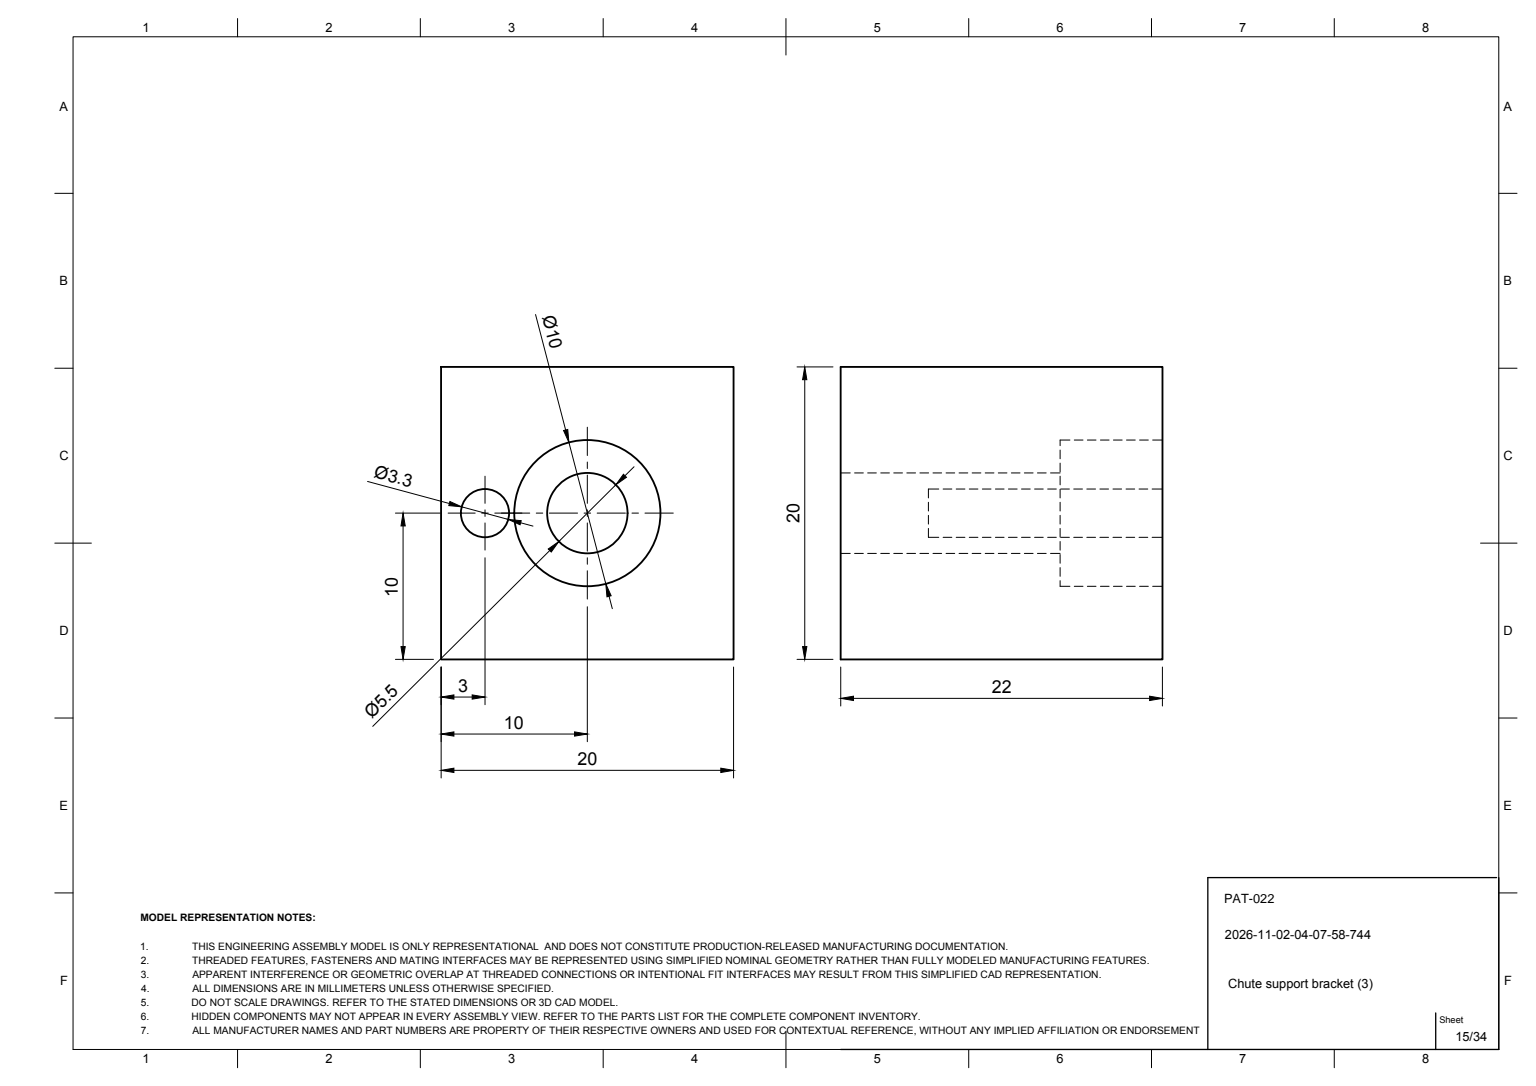
ISO-10303-21;
HEADER;
/* Generated by software containing ST-Developer
 * from STEP Tools, Inc. (www.steptools.com) 
 */

FILE_DESCRIPTION(
/* description */ ('Chute with adjustable gate'),
/* implementation_level */ '2;1');

FILE_NAME(
/* name */ 'Chute support bracket (3).step',
/* time_stamp */ '2026-10-27T10:52:28-07:00',
/* author */ (''),
/* organization */ (''),
/* preprocessor_version */ 'ST-DEVELOPER v20.2',
/* originating_system */ 'Autodesk Translation Framework v15.17.0.0',
/* authorisation */ '');

FILE_SCHEMA (('AUTOMOTIVE_DESIGN { 1 0 10303 214 3 1 1 }'));
ENDSEC;

DATA;
#10=MECHANICAL_DESIGN_GEOMETRIC_PRESENTATION_REPRESENTATION('',(#424),#13094);
#360=SHAPE_REPRESENTATION_RELATIONSHIP('SRR','None',#13261,#392);
#392=ADVANCED_BREP_SHAPE_REPRESENTATION('',(#456),#13070);
#424=STYLED_ITEM('',(#13474),#456);
#456=MANIFOLD_SOLID_BREP('Body1',#7607);
#512=FACE_BOUND('',#1462,.T.);
#513=FACE_BOUND('',#1465,.T.);
#514=FACE_BOUND('',#1468,.T.);
#515=FACE_BOUND('',#1469,.T.);
#660=PLANE('',#8135);
#661=PLANE('',#8139);
#662=PLANE('',#8143);
#663=PLANE('',#8144);
#664=PLANE('',#8145);
#665=PLANE('',#8146);
#666=PLANE('',#8147);
#667=PLANE('',#8148);
#1005=FACE_OUTER_BOUND('',#1458,.T.);
#1006=FACE_OUTER_BOUND('',#1459,.T.);
#1007=FACE_OUTER_BOUND('',#1460,.T.);
#1008=FACE_OUTER_BOUND('',#1461,.T.);
#1009=FACE_OUTER_BOUND('',#1463,.T.);
#1010=FACE_OUTER_BOUND('',#1464,.T.);
#1011=FACE_OUTER_BOUND('',#1466,.T.);
#1012=FACE_OUTER_BOUND('',#1467,.T.);
#1013=FACE_OUTER_BOUND('',#1470,.T.);
#1014=FACE_OUTER_BOUND('',#1471,.T.);
#1015=FACE_OUTER_BOUND('',#1472,.T.);
#1458=EDGE_LOOP('',(#5576,#5577,#5578,#5579));
#1459=EDGE_LOOP('',(#5580));
#1460=EDGE_LOOP('',(#5581,#5582,#5583,#5584));
#1461=EDGE_LOOP('',(#5585));
#1462=EDGE_LOOP('',(#5586));
#1463=EDGE_LOOP('',(#5587,#5588,#5589,#5590));
#1464=EDGE_LOOP('',(#5591,#5592,#5593,#5594));
#1465=EDGE_LOOP('',(#5595));
#1466=EDGE_LOOP('',(#5596,#5597,#5598,#5599));
#1467=EDGE_LOOP('',(#5600,#5601,#5602,#5603));
#1468=EDGE_LOOP('',(#5604));
#1469=EDGE_LOOP('',(#5605));
#1470=EDGE_LOOP('',(#5606,#5607,#5608,#5609));
#1471=EDGE_LOOP('',(#5610,#5611,#5612,#5613));
#1472=EDGE_LOOP('',(#5614,#5615,#5616,#5617));
#2013=LINE('',#11332,#2790);
#2014=LINE('',#11339,#2791);
#2015=LINE('',#11346,#2792);
#2016=LINE('',#11351,#2793);
#2017=LINE('',#11353,#2794);
#2018=LINE('',#11355,#2795);
#2019=LINE('',#11356,#2796);
#2020=LINE('',#11359,#2797);
#2021=LINE('',#11361,#2798);
#2022=LINE('',#11362,#2799);
#2023=LINE('',#11365,#2800);
#2024=LINE('',#11367,#2801);
#2025=LINE('',#11368,#2802);
#2026=LINE('',#11370,#2803);
#2027=LINE('',#11371,#2804);
#2790=VECTOR('',#9147,0.164999999999999);
#2791=VECTOR('',#9156,0.5);
#2792=VECTOR('',#9165,0.274999999999999);
#2793=VECTOR('',#9170,1.);
#2794=VECTOR('',#9171,1.);
#2795=VECTOR('',#9172,1.);
#2796=VECTOR('',#9173,1.);
#2797=VECTOR('',#9176,1.);
#2798=VECTOR('',#9177,1.);
#2799=VECTOR('',#9178,1.);
#2800=VECTOR('',#9181,1.);
#2801=VECTOR('',#9182,1.);
#2802=VECTOR('',#9183,1.);
#2803=VECTOR('',#9186,1.);
#2804=VECTOR('',#9187,1.);
#3456=CIRCLE('',#8133,0.164999999999999);
#3457=CIRCLE('',#8134,0.164999999999999);
#3458=CIRCLE('',#8137,0.5);
#3459=CIRCLE('',#8138,0.5);
#3460=CIRCLE('',#8140,0.274999999999999);
#3461=CIRCLE('',#8142,0.274999999999999);
#3723=VERTEX_POINT('',#11329);
#3724=VERTEX_POINT('',#11331);
#3725=VERTEX_POINT('',#11336);
#3726=VERTEX_POINT('',#11338);
#3727=VERTEX_POINT('',#11342);
#3728=VERTEX_POINT('',#11345);
#3729=VERTEX_POINT('',#11349);
#3730=VERTEX_POINT('',#11350);
#3731=VERTEX_POINT('',#11352);
#3732=VERTEX_POINT('',#11354);
#3733=VERTEX_POINT('',#11358);
#3734=VERTEX_POINT('',#11360);
#3735=VERTEX_POINT('',#11364);
#3736=VERTEX_POINT('',#11366);
#4421=EDGE_CURVE('',#3723,#3723,#3456,.T.);
#4422=EDGE_CURVE('',#3723,#3724,#2013,.T.);
#4423=EDGE_CURVE('',#3724,#3724,#3457,.T.);
#4424=EDGE_CURVE('',#3725,#3725,#3458,.T.);
#4425=EDGE_CURVE('',#3725,#3726,#2014,.T.);
#4426=EDGE_CURVE('',#3726,#3726,#3459,.T.);
#4427=EDGE_CURVE('',#3727,#3727,#3460,.T.);
#4428=EDGE_CURVE('',#3727,#3728,#2015,.T.);
#4429=EDGE_CURVE('',#3728,#3728,#3461,.T.);
#4430=EDGE_CURVE('',#3729,#3730,#2016,.T.);
#4431=EDGE_CURVE('',#3730,#3731,#2017,.T.);
#4432=EDGE_CURVE('',#3732,#3731,#2018,.T.);
#4433=EDGE_CURVE('',#3729,#3732,#2019,.T.);
#4434=EDGE_CURVE('',#3733,#3729,#2020,.T.);
#4435=EDGE_CURVE('',#3734,#3732,#2021,.T.);
#4436=EDGE_CURVE('',#3733,#3734,#2022,.T.);
#4437=EDGE_CURVE('',#3735,#3733,#2023,.T.);
#4438=EDGE_CURVE('',#3736,#3734,#2024,.T.);
#4439=EDGE_CURVE('',#3735,#3736,#2025,.T.);
#4440=EDGE_CURVE('',#3730,#3735,#2026,.T.);
#4441=EDGE_CURVE('',#3731,#3736,#2027,.T.);
#5576=ORIENTED_EDGE('',*,*,#4421,.F.);
#5577=ORIENTED_EDGE('',*,*,#4422,.T.);
#5578=ORIENTED_EDGE('',*,*,#4423,.T.);
#5579=ORIENTED_EDGE('',*,*,#4422,.F.);
#5580=ORIENTED_EDGE('',*,*,#4423,.F.);
#5581=ORIENTED_EDGE('',*,*,#4424,.F.);
#5582=ORIENTED_EDGE('',*,*,#4425,.T.);
#5583=ORIENTED_EDGE('',*,*,#4426,.T.);
#5584=ORIENTED_EDGE('',*,*,#4425,.F.);
#5585=ORIENTED_EDGE('',*,*,#4426,.F.);
#5586=ORIENTED_EDGE('',*,*,#4427,.F.);
#5587=ORIENTED_EDGE('',*,*,#4427,.T.);
#5588=ORIENTED_EDGE('',*,*,#4428,.T.);
#5589=ORIENTED_EDGE('',*,*,#4429,.F.);
#5590=ORIENTED_EDGE('',*,*,#4428,.F.);
#5591=ORIENTED_EDGE('',*,*,#4430,.T.);
#5592=ORIENTED_EDGE('',*,*,#4431,.T.);
#5593=ORIENTED_EDGE('',*,*,#4432,.F.);
#5594=ORIENTED_EDGE('',*,*,#4433,.F.);
#5595=ORIENTED_EDGE('',*,*,#4429,.T.);
#5596=ORIENTED_EDGE('',*,*,#4434,.T.);
#5597=ORIENTED_EDGE('',*,*,#4433,.T.);
#5598=ORIENTED_EDGE('',*,*,#4435,.F.);
#5599=ORIENTED_EDGE('',*,*,#4436,.F.);
#5600=ORIENTED_EDGE('',*,*,#4437,.T.);
#5601=ORIENTED_EDGE('',*,*,#4436,.T.);
#5602=ORIENTED_EDGE('',*,*,#4438,.F.);
#5603=ORIENTED_EDGE('',*,*,#4439,.F.);
#5604=ORIENTED_EDGE('',*,*,#4421,.T.);
#5605=ORIENTED_EDGE('',*,*,#4424,.T.);
#5606=ORIENTED_EDGE('',*,*,#4440,.T.);
#5607=ORIENTED_EDGE('',*,*,#4439,.T.);
#5608=ORIENTED_EDGE('',*,*,#4441,.F.);
#5609=ORIENTED_EDGE('',*,*,#4431,.F.);
#5610=ORIENTED_EDGE('',*,*,#4441,.T.);
#5611=ORIENTED_EDGE('',*,*,#4438,.T.);
#5612=ORIENTED_EDGE('',*,*,#4435,.T.);
#5613=ORIENTED_EDGE('',*,*,#4432,.T.);
#5614=ORIENTED_EDGE('',*,*,#4440,.F.);
#5615=ORIENTED_EDGE('',*,*,#4430,.F.);
#5616=ORIENTED_EDGE('',*,*,#4434,.F.);
#5617=ORIENTED_EDGE('',*,*,#4437,.F.);
#7127=CYLINDRICAL_SURFACE('',#8132,0.164999999999999);
#7128=CYLINDRICAL_SURFACE('',#8136,0.5);
#7129=CYLINDRICAL_SURFACE('',#8141,0.274999999999999);
#7273=ADVANCED_FACE('',(#1005),#7127,.F.);
#7274=ADVANCED_FACE('',(#1006),#660,.F.);
#7275=ADVANCED_FACE('',(#1007),#7128,.F.);
#7276=ADVANCED_FACE('',(#1008,#512),#661,.F.);
#7277=ADVANCED_FACE('',(#1009),#7129,.F.);
#7278=ADVANCED_FACE('',(#1010,#513),#662,.T.);
#7279=ADVANCED_FACE('',(#1011),#663,.T.);
#7280=ADVANCED_FACE('',(#1012,#514,#515),#664,.T.);
#7281=ADVANCED_FACE('',(#1013),#665,.T.);
#7282=ADVANCED_FACE('',(#1014),#666,.T.);
#7283=ADVANCED_FACE('',(#1015),#667,.F.);
#7607=CLOSED_SHELL('',(#7273,#7274,#7275,#7276,#7277,#7278,#7279,#7280,
#7281,#7282,#7283));
#8131=AXIS2_PLACEMENT_3D('',#11327,#9141,#9142);
#8132=AXIS2_PLACEMENT_3D('',#11328,#9143,#9144);
#8133=AXIS2_PLACEMENT_3D('',#11330,#9145,#9146);
#8134=AXIS2_PLACEMENT_3D('',#11333,#9148,#9149);
#8135=AXIS2_PLACEMENT_3D('',#11334,#9150,#9151);
#8136=AXIS2_PLACEMENT_3D('',#11335,#9152,#9153);
#8137=AXIS2_PLACEMENT_3D('',#11337,#9154,#9155);
#8138=AXIS2_PLACEMENT_3D('',#11340,#9157,#9158);
#8139=AXIS2_PLACEMENT_3D('',#11341,#9159,#9160);
#8140=AXIS2_PLACEMENT_3D('',#11343,#9161,#9162);
#8141=AXIS2_PLACEMENT_3D('',#11344,#9163,#9164);
#8142=AXIS2_PLACEMENT_3D('',#11347,#9166,#9167);
#8143=AXIS2_PLACEMENT_3D('',#11348,#9168,#9169);
#8144=AXIS2_PLACEMENT_3D('',#11357,#9174,#9175);
#8145=AXIS2_PLACEMENT_3D('',#11363,#9179,#9180);
#8146=AXIS2_PLACEMENT_3D('',#11369,#9184,#9185);
#8147=AXIS2_PLACEMENT_3D('',#11372,#9188,#9189);
#8148=AXIS2_PLACEMENT_3D('',#11373,#9190,#9191);
#9141=DIRECTION('axis',(0.,0.,1.));
#9142=DIRECTION('refdir',(1.,0.,0.));
#9143=DIRECTION('center_axis',(0.,1.,0.));
#9144=DIRECTION('ref_axis',(1.,0.,0.));
#9145=DIRECTION('center_axis',(0.,1.,0.));
#9146=DIRECTION('ref_axis',(1.,0.,0.));
#9147=DIRECTION('',(0.,1.,0.));
#9148=DIRECTION('center_axis',(0.,1.,0.));
#9149=DIRECTION('ref_axis',(1.,0.,0.));
#9150=DIRECTION('center_axis',(0.,1.,0.));
#9151=DIRECTION('ref_axis',(1.,0.,0.));
#9152=DIRECTION('center_axis',(0.,1.,0.));
#9153=DIRECTION('ref_axis',(1.,0.,0.));
#9154=DIRECTION('center_axis',(0.,1.,0.));
#9155=DIRECTION('ref_axis',(1.,0.,0.));
#9156=DIRECTION('',(0.,1.,0.));
#9157=DIRECTION('center_axis',(0.,1.,0.));
#9158=DIRECTION('ref_axis',(1.,0.,0.));
#9159=DIRECTION('center_axis',(0.,1.,0.));
#9160=DIRECTION('ref_axis',(1.,0.,0.));
#9161=DIRECTION('center_axis',(0.,-1.,0.));
#9162=DIRECTION('ref_axis',(1.,0.,0.));
#9163=DIRECTION('center_axis',(0.,1.,0.));
#9164=DIRECTION('ref_axis',(1.,0.,0.));
#9165=DIRECTION('',(0.,1.,0.));
#9166=DIRECTION('center_axis',(0.,-1.,0.));
#9167=DIRECTION('ref_axis',(1.,0.,0.));
#9168=DIRECTION('center_axis',(0.,1.,0.));
#9169=DIRECTION('ref_axis',(-1.,0.,0.));
#9170=DIRECTION('',(-1.,0.,0.));
#9171=DIRECTION('',(0.,0.,1.));
#9172=DIRECTION('',(-1.,0.,0.));
#9173=DIRECTION('',(0.,0.,1.));
#9174=DIRECTION('center_axis',(1.,0.,0.));
#9175=DIRECTION('ref_axis',(0.,1.,0.));
#9176=DIRECTION('',(0.,1.,0.));
#9177=DIRECTION('',(0.,1.,0.));
#9178=DIRECTION('',(0.,0.,1.));
#9179=DIRECTION('center_axis',(0.,-1.,0.));
#9180=DIRECTION('ref_axis',(1.,0.,0.));
#9181=DIRECTION('',(1.,0.,0.));
#9182=DIRECTION('',(1.,0.,0.));
#9183=DIRECTION('',(0.,0.,1.));
#9184=DIRECTION('center_axis',(-1.,0.,0.));
#9185=DIRECTION('ref_axis',(0.,-1.,0.));
#9186=DIRECTION('',(0.,-1.,0.));
#9187=DIRECTION('',(0.,-1.,0.));
#9188=DIRECTION('center_axis',(0.,0.,1.));
#9189=DIRECTION('ref_axis',(1.,0.,0.));
#9190=DIRECTION('center_axis',(0.,0.,1.));
#9191=DIRECTION('ref_axis',(1.,0.,0.));
#11327=CARTESIAN_POINT('',(0.,0.,0.));
#11328=CARTESIAN_POINT('Origin',(22.3,7.7,12.));
#11329=CARTESIAN_POINT('',(22.135,7.8,12.));
#11330=CARTESIAN_POINT('Origin',(22.3,7.8,12.));
#11331=CARTESIAN_POINT('',(22.135,9.4,12.));
#11332=CARTESIAN_POINT('',(22.135,7.7,12.));
#11333=CARTESIAN_POINT('Origin',(22.3,9.4,12.));
#11334=CARTESIAN_POINT('Origin',(22.3,9.4,12.));
#11335=CARTESIAN_POINT('Origin',(23.,7.7,12.));
#11336=CARTESIAN_POINT('',(22.5,7.8,12.));
#11337=CARTESIAN_POINT('Origin',(23.,7.8,12.));
#11338=CARTESIAN_POINT('',(22.5,8.5,12.));
#11339=CARTESIAN_POINT('',(22.5,7.7,12.));
#11340=CARTESIAN_POINT('Origin',(23.,8.5,12.));
#11341=CARTESIAN_POINT('Origin',(23.,8.5,12.));
#11342=CARTESIAN_POINT('',(22.725,8.5,12.));
#11343=CARTESIAN_POINT('Origin',(23.,8.5,12.));
#11344=CARTESIAN_POINT('Origin',(23.,7.7,12.));
#11345=CARTESIAN_POINT('',(22.725,10.,12.));
#11346=CARTESIAN_POINT('',(22.725,7.7,12.));
#11347=CARTESIAN_POINT('Origin',(23.,10.,12.));
#11348=CARTESIAN_POINT('Origin',(24.,10.,11.));
#11349=CARTESIAN_POINT('',(24.,10.,11.));
#11350=CARTESIAN_POINT('',(22.,10.,11.));
#11351=CARTESIAN_POINT('',(24.,10.,11.));
#11352=CARTESIAN_POINT('',(22.,10.,13.));
#11353=CARTESIAN_POINT('',(22.,10.,11.));
#11354=CARTESIAN_POINT('',(24.,10.,13.));
#11355=CARTESIAN_POINT('',(24.,10.,13.));
#11356=CARTESIAN_POINT('',(24.,10.,11.));
#11357=CARTESIAN_POINT('Origin',(24.,7.8,11.));
#11358=CARTESIAN_POINT('',(24.,7.8,11.));
#11359=CARTESIAN_POINT('',(24.,7.8,11.));
#11360=CARTESIAN_POINT('',(24.,7.8,13.));
#11361=CARTESIAN_POINT('',(24.,7.8,13.));
#11362=CARTESIAN_POINT('',(24.,7.8,11.));
#11363=CARTESIAN_POINT('Origin',(22.,7.8,11.));
#11364=CARTESIAN_POINT('',(22.,7.8,11.));
#11365=CARTESIAN_POINT('',(22.,7.8,11.));
#11366=CARTESIAN_POINT('',(22.,7.8,13.));
#11367=CARTESIAN_POINT('',(22.,7.8,13.));
#11368=CARTESIAN_POINT('',(22.,7.8,11.));
#11369=CARTESIAN_POINT('Origin',(22.,10.,11.));
#11370=CARTESIAN_POINT('',(22.,10.,11.));
#11371=CARTESIAN_POINT('',(22.,10.,13.));
#11372=CARTESIAN_POINT('Origin',(23.,8.9,13.));
#11373=CARTESIAN_POINT('Origin',(23.,8.9,11.));
#13033=UNCERTAINTY_MEASURE_WITH_UNIT(LENGTH_MEASURE(0.001),#13095,
'DISTANCE_ACCURACY_VALUE',
'Maximum model space distance between geometric entities at asserted c
onnectivities');
#13057=UNCERTAINTY_MEASURE_WITH_UNIT(LENGTH_MEASURE(0.001),#13095,
'DISTANCE_ACCURACY_VALUE',
'Maximum model space distance between geometric entities at asserted c
onnectivities');
#13070=(
GEOMETRIC_REPRESENTATION_CONTEXT(3)
GLOBAL_UNCERTAINTY_ASSIGNED_CONTEXT((#13033))
GLOBAL_UNIT_ASSIGNED_CONTEXT((#13095,#13097,#13098))
REPRESENTATION_CONTEXT('','3D')
);
#13094=(
GEOMETRIC_REPRESENTATION_CONTEXT(3)
GLOBAL_UNCERTAINTY_ASSIGNED_CONTEXT((#13057))
GLOBAL_UNIT_ASSIGNED_CONTEXT((#13095,#13097,#13098))
REPRESENTATION_CONTEXT('','3D')
);
#13095=(
LENGTH_UNIT()
NAMED_UNIT(*)
SI_UNIT(.CENTI.,.METRE.)
);
#13097=(
NAMED_UNIT(*)
PLANE_ANGLE_UNIT()
SI_UNIT($,.RADIAN.)
);
#13098=(
NAMED_UNIT(*)
SI_UNIT($,.STERADIAN.)
SOLID_ANGLE_UNIT()
);
#13111=SHAPE_DEFINITION_REPRESENTATION(#13147,#13261);
#13147=PRODUCT_DEFINITION_SHAPE('',$,#13298);
#13261=SHAPE_REPRESENTATION('',(#8131),#13070);
#13285=PRODUCT_DEFINITION_CONTEXT('part definition',#13395,'design');
#13298=PRODUCT_DEFINITION('Chute support bracket (3)',
'Chute support bracket (3)',#13334,#13285);
#13334=PRODUCT_DEFINITION_FORMATION('',$,#13409);
#13395=APPLICATION_CONTEXT(
'Core Data for Automotive Mechanical Design Process');
#13396=PRODUCT_CONTEXT('part definition',#13395,'mechanical');
#13409=PRODUCT('Chute support bracket (3)','Chute support bracket (3)',
'Chute support bracket (3)',(#13396));
#13468=COLOUR_RGB('Dark Blue',0.08,0.2,0.34);
#13469=FILL_AREA_STYLE_COLOUR('',#13468);
#13470=FILL_AREA_STYLE('',(#13469));
#13471=SURFACE_STYLE_FILL_AREA(#13470);
#13472=SURFACE_SIDE_STYLE('',(#13471));
#13473=SURFACE_STYLE_USAGE(.BOTH.,#13472);
#13474=PRESENTATION_STYLE_ASSIGNMENT((#13473));
ENDSEC;
END-ISO-10303-21;
